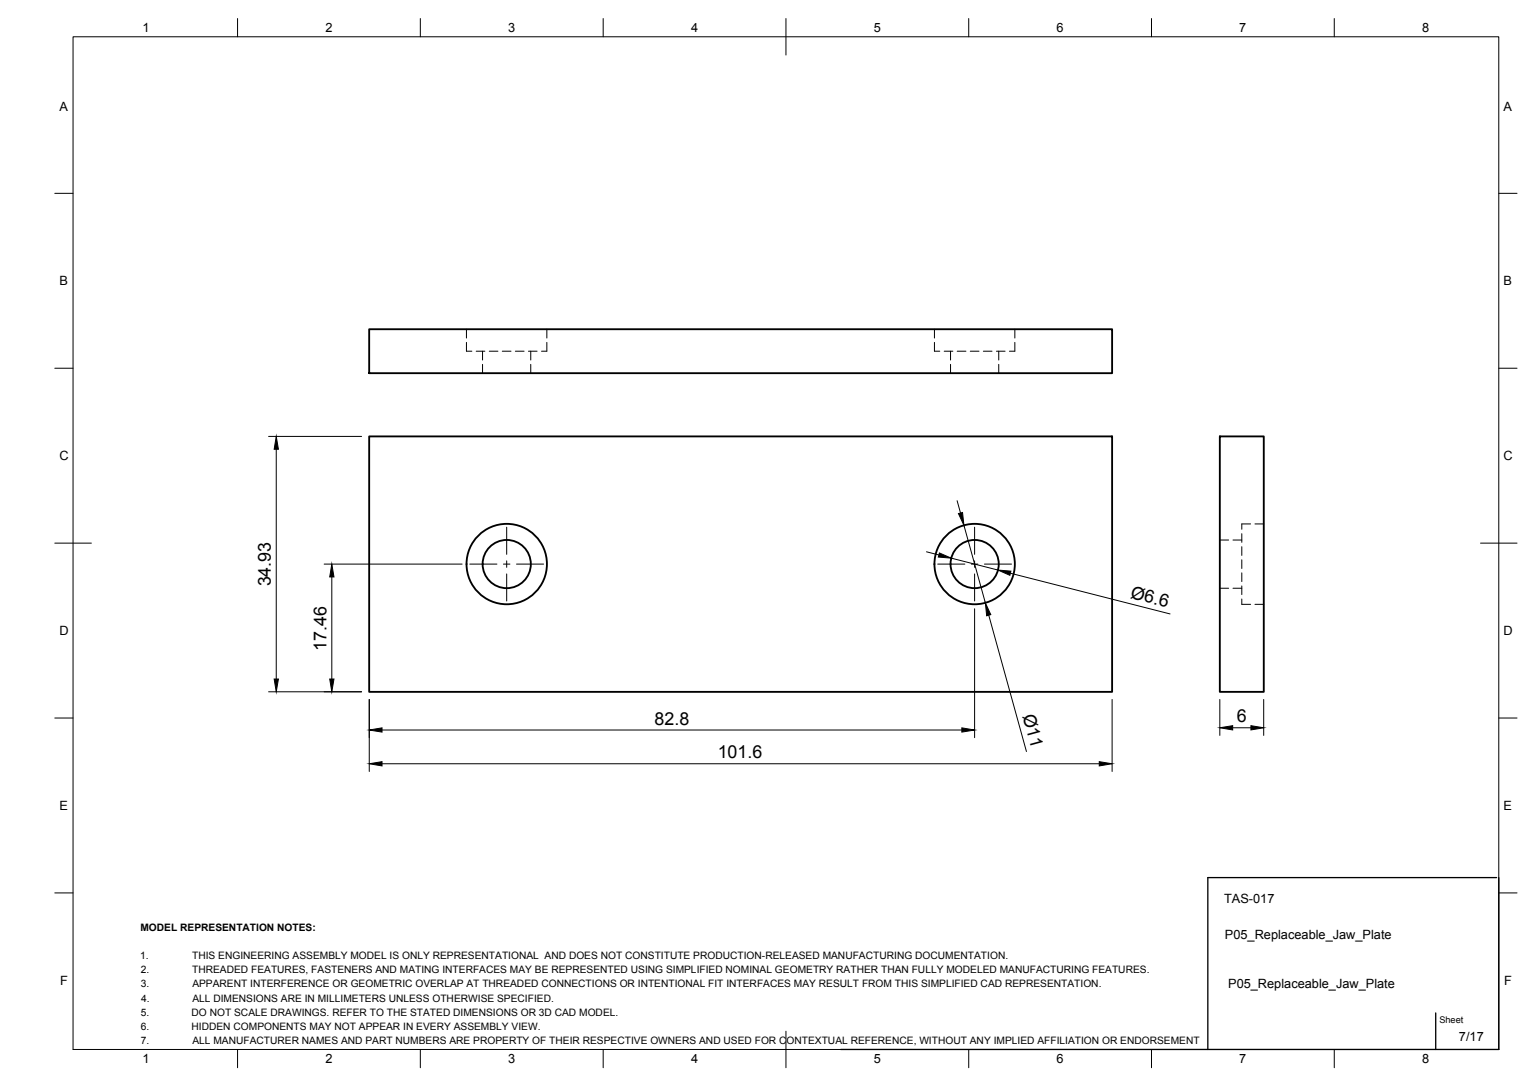
ISO-10303-21;
HEADER;
/* Generated by software containing ST-Developer
 * from STEP Tools, Inc. (www.steptools.com) 
 */

FILE_DESCRIPTION(
/* description */ ('STEP AP203'),
/* implementation_level */ '2;1');

FILE_NAME(
/* name */ 'P05_Replaceable_Jaw_Plate.step',
/* time_stamp */ '2026-11-15T15:04:01-08:00',
/* author */ (''),
/* organization */ (''),
/* preprocessor_version */ 'ST-DEVELOPER v20.2',
/* originating_system */ 'Autodesk Translation Framework v15.17.0.0',
/* authorisation */ '');

FILE_SCHEMA (('AUTOMOTIVE_DESIGN { 1 0 10303 214 3 1 1 }'));
ENDSEC;

DATA;
#10=MECHANICAL_DESIGN_GEOMETRIC_PRESENTATION_REPRESENTATION('',(#296),#16598);
#218=SHAPE_REPRESENTATION_RELATIONSHIP('SRR','None',#16712,#242);
#242=ADVANCED_BREP_SHAPE_REPRESENTATION('',(#266),#16588);
#266=MANIFOLD_SOLID_BREP('Body1',#9801);
#296=STYLED_ITEM('',(#16834),#266);
#362=FACE_BOUND('',#1777,.T.);
#363=FACE_BOUND('',#1778,.T.);
#364=FACE_BOUND('',#1780,.T.);
#365=FACE_BOUND('',#1781,.T.);
#366=FACE_BOUND('',#1783,.T.);
#367=FACE_BOUND('',#1785,.T.);
#633=PLANE('',#10459);
#634=PLANE('',#10460);
#635=PLANE('',#10461);
#636=PLANE('',#10462);
#637=PLANE('',#10463);
#638=PLANE('',#10464);
#639=PLANE('',#10465);
#640=PLANE('',#10466);
#1161=FACE_OUTER_BOUND('',#1768,.T.);
#1162=FACE_OUTER_BOUND('',#1769,.T.);
#1163=FACE_OUTER_BOUND('',#1770,.T.);
#1164=FACE_OUTER_BOUND('',#1771,.T.);
#1165=FACE_OUTER_BOUND('',#1772,.T.);
#1166=FACE_OUTER_BOUND('',#1773,.T.);
#1167=FACE_OUTER_BOUND('',#1774,.T.);
#1168=FACE_OUTER_BOUND('',#1775,.T.);
#1169=FACE_OUTER_BOUND('',#1776,.T.);
#1170=FACE_OUTER_BOUND('',#1779,.T.);
#1171=FACE_OUTER_BOUND('',#1782,.T.);
#1172=FACE_OUTER_BOUND('',#1784,.T.);
#1768=EDGE_LOOP('',(#7767,#7768,#7769,#7770));
#1769=EDGE_LOOP('',(#7771,#7772,#7773,#7774));
#1770=EDGE_LOOP('',(#7775,#7776,#7777,#7778));
#1771=EDGE_LOOP('',(#7779,#7780,#7781,#7782));
#1772=EDGE_LOOP('',(#7783,#7784,#7785,#7786));
#1773=EDGE_LOOP('',(#7787,#7788,#7789,#7790));
#1774=EDGE_LOOP('',(#7791,#7792,#7793,#7794));
#1775=EDGE_LOOP('',(#7795,#7796,#7797,#7798));
#1776=EDGE_LOOP('',(#7799,#7800,#7801,#7802));
#1777=EDGE_LOOP('',(#7803));
#1778=EDGE_LOOP('',(#7804));
#1779=EDGE_LOOP('',(#7805,#7806,#7807,#7808));
#1780=EDGE_LOOP('',(#7809));
#1781=EDGE_LOOP('',(#7810));
#1782=EDGE_LOOP('',(#7811));
#1783=EDGE_LOOP('',(#7812));
#1784=EDGE_LOOP('',(#7813));
#1785=EDGE_LOOP('',(#7814));
#2610=LINE('',#15029,#3658);
#2611=LINE('',#15035,#3659);
#2612=LINE('',#15041,#3660);
#2613=LINE('',#15047,#3661);
#2614=LINE('',#15052,#3662);
#2615=LINE('',#15054,#3663);
#2616=LINE('',#15056,#3664);
#2617=LINE('',#15057,#3665);
#2618=LINE('',#15060,#3666);
#2619=LINE('',#15062,#3667);
#2620=LINE('',#15063,#3668);
#2621=LINE('',#15066,#3669);
#2622=LINE('',#15068,#3670);
#2623=LINE('',#15069,#3671);
#2624=LINE('',#15071,#3672);
#2625=LINE('',#15072,#3673);
#3658=VECTOR('',#12148,5.50000000000001);
#3659=VECTOR('',#12155,5.50000000000001);
#3660=VECTOR('',#12162,3.3);
#3661=VECTOR('',#12169,3.3);
#3662=VECTOR('',#12174,1000.);
#3663=VECTOR('',#12175,1000.);
#3664=VECTOR('',#12176,1000.);
#3665=VECTOR('',#12177,1000.);
#3666=VECTOR('',#12180,1000.);
#3667=VECTOR('',#12181,1000.);
#3668=VECTOR('',#12182,1000.);
#3669=VECTOR('',#12185,1000.);
#3670=VECTOR('',#12186,1000.);
#3671=VECTOR('',#12187,1000.);
#3672=VECTOR('',#12190,1000.);
#3673=VECTOR('',#12191,1000.);
#4328=CIRCLE('',#10448,5.50000000000001);
#4329=CIRCLE('',#10449,5.50000000000001);
#4330=CIRCLE('',#10451,5.50000000000001);
#4331=CIRCLE('',#10452,5.50000000000001);
#4332=CIRCLE('',#10454,3.3);
#4333=CIRCLE('',#10455,3.3);
#4334=CIRCLE('',#10457,3.3);
#4335=CIRCLE('',#10458,3.3);
#4844=VERTEX_POINT('',#15026);
#4845=VERTEX_POINT('',#15028);
#4846=VERTEX_POINT('',#15032);
#4847=VERTEX_POINT('',#15034);
#4848=VERTEX_POINT('',#15038);
#4849=VERTEX_POINT('',#15040);
#4850=VERTEX_POINT('',#15044);
#4851=VERTEX_POINT('',#15046);
#4852=VERTEX_POINT('',#15050);
#4853=VERTEX_POINT('',#15051);
#4854=VERTEX_POINT('',#15053);
#4855=VERTEX_POINT('',#15055);
#4856=VERTEX_POINT('',#15059);
#4857=VERTEX_POINT('',#15061);
#4858=VERTEX_POINT('',#15065);
#4859=VERTEX_POINT('',#15067);
#5896=EDGE_CURVE('',#4844,#4844,#4328,.T.);
#5897=EDGE_CURVE('',#4844,#4845,#2610,.T.);
#5898=EDGE_CURVE('',#4845,#4845,#4329,.T.);
#5899=EDGE_CURVE('',#4846,#4846,#4330,.T.);
#5900=EDGE_CURVE('',#4846,#4847,#2611,.T.);
#5901=EDGE_CURVE('',#4847,#4847,#4331,.T.);
#5902=EDGE_CURVE('',#4848,#4848,#4332,.T.);
#5903=EDGE_CURVE('',#4848,#4849,#2612,.T.);
#5904=EDGE_CURVE('',#4849,#4849,#4333,.T.);
#5905=EDGE_CURVE('',#4850,#4850,#4334,.T.);
#5906=EDGE_CURVE('',#4850,#4851,#2613,.T.);
#5907=EDGE_CURVE('',#4851,#4851,#4335,.T.);
#5908=EDGE_CURVE('',#4852,#4853,#2614,.T.);
#5909=EDGE_CURVE('',#4854,#4853,#2615,.T.);
#5910=EDGE_CURVE('',#4855,#4854,#2616,.T.);
#5911=EDGE_CURVE('',#4855,#4852,#2617,.T.);
#5912=EDGE_CURVE('',#4853,#4856,#2618,.T.);
#5913=EDGE_CURVE('',#4857,#4856,#2619,.T.);
#5914=EDGE_CURVE('',#4854,#4857,#2620,.T.);
#5915=EDGE_CURVE('',#4856,#4858,#2621,.T.);
#5916=EDGE_CURVE('',#4859,#4858,#2622,.T.);
#5917=EDGE_CURVE('',#4857,#4859,#2623,.T.);
#5918=EDGE_CURVE('',#4858,#4852,#2624,.T.);
#5919=EDGE_CURVE('',#4859,#4855,#2625,.T.);
#7767=ORIENTED_EDGE('',*,*,#5896,.T.);
#7768=ORIENTED_EDGE('',*,*,#5897,.T.);
#7769=ORIENTED_EDGE('',*,*,#5898,.F.);
#7770=ORIENTED_EDGE('',*,*,#5897,.F.);
#7771=ORIENTED_EDGE('',*,*,#5899,.T.);
#7772=ORIENTED_EDGE('',*,*,#5900,.T.);
#7773=ORIENTED_EDGE('',*,*,#5901,.F.);
#7774=ORIENTED_EDGE('',*,*,#5900,.F.);
#7775=ORIENTED_EDGE('',*,*,#5902,.F.);
#7776=ORIENTED_EDGE('',*,*,#5903,.T.);
#7777=ORIENTED_EDGE('',*,*,#5904,.F.);
#7778=ORIENTED_EDGE('',*,*,#5903,.F.);
#7779=ORIENTED_EDGE('',*,*,#5905,.F.);
#7780=ORIENTED_EDGE('',*,*,#5906,.T.);
#7781=ORIENTED_EDGE('',*,*,#5907,.F.);
#7782=ORIENTED_EDGE('',*,*,#5906,.F.);
#7783=ORIENTED_EDGE('',*,*,#5908,.T.);
#7784=ORIENTED_EDGE('',*,*,#5909,.F.);
#7785=ORIENTED_EDGE('',*,*,#5910,.F.);
#7786=ORIENTED_EDGE('',*,*,#5911,.T.);
#7787=ORIENTED_EDGE('',*,*,#5912,.T.);
#7788=ORIENTED_EDGE('',*,*,#5913,.F.);
#7789=ORIENTED_EDGE('',*,*,#5914,.F.);
#7790=ORIENTED_EDGE('',*,*,#5909,.T.);
#7791=ORIENTED_EDGE('',*,*,#5915,.T.);
#7792=ORIENTED_EDGE('',*,*,#5916,.F.);
#7793=ORIENTED_EDGE('',*,*,#5917,.F.);
#7794=ORIENTED_EDGE('',*,*,#5913,.T.);
#7795=ORIENTED_EDGE('',*,*,#5918,.T.);
#7796=ORIENTED_EDGE('',*,*,#5911,.F.);
#7797=ORIENTED_EDGE('',*,*,#5919,.F.);
#7798=ORIENTED_EDGE('',*,*,#5916,.T.);
#7799=ORIENTED_EDGE('',*,*,#5910,.T.);
#7800=ORIENTED_EDGE('',*,*,#5914,.T.);
#7801=ORIENTED_EDGE('',*,*,#5917,.T.);
#7802=ORIENTED_EDGE('',*,*,#5919,.T.);
#7803=ORIENTED_EDGE('',*,*,#5902,.T.);
#7804=ORIENTED_EDGE('',*,*,#5905,.T.);
#7805=ORIENTED_EDGE('',*,*,#5908,.F.);
#7806=ORIENTED_EDGE('',*,*,#5918,.F.);
#7807=ORIENTED_EDGE('',*,*,#5915,.F.);
#7808=ORIENTED_EDGE('',*,*,#5912,.F.);
#7809=ORIENTED_EDGE('',*,*,#5901,.T.);
#7810=ORIENTED_EDGE('',*,*,#5898,.T.);
#7811=ORIENTED_EDGE('',*,*,#5899,.F.);
#7812=ORIENTED_EDGE('',*,*,#5904,.T.);
#7813=ORIENTED_EDGE('',*,*,#5896,.F.);
#7814=ORIENTED_EDGE('',*,*,#5907,.T.);
#9215=CYLINDRICAL_SURFACE('',#10447,5.50000000000001);
#9216=CYLINDRICAL_SURFACE('',#10450,5.50000000000001);
#9217=CYLINDRICAL_SURFACE('',#10453,3.3);
#9218=CYLINDRICAL_SURFACE('',#10456,3.3);
#9486=ADVANCED_FACE('',(#1161),#9215,.F.);
#9487=ADVANCED_FACE('',(#1162),#9216,.F.);
#9488=ADVANCED_FACE('',(#1163),#9217,.F.);
#9489=ADVANCED_FACE('',(#1164),#9218,.F.);
#9490=ADVANCED_FACE('',(#1165),#633,.F.);
#9491=ADVANCED_FACE('',(#1166),#634,.F.);
#9492=ADVANCED_FACE('',(#1167),#635,.F.);
#9493=ADVANCED_FACE('',(#1168),#636,.F.);
#9494=ADVANCED_FACE('',(#1169,#362,#363),#637,.T.);
#9495=ADVANCED_FACE('',(#1170,#364,#365),#638,.F.);
#9496=ADVANCED_FACE('',(#1171,#366),#639,.F.);
#9497=ADVANCED_FACE('',(#1172,#367),#640,.F.);
#9801=CLOSED_SHELL('',(#9486,#9487,#9488,#9489,#9490,#9491,#9492,#9493,
#9494,#9495,#9496,#9497));
#10446=AXIS2_PLACEMENT_3D('',#15024,#12142,#12143);
#10447=AXIS2_PLACEMENT_3D('',#15025,#12144,#12145);
#10448=AXIS2_PLACEMENT_3D('',#15027,#12146,#12147);
#10449=AXIS2_PLACEMENT_3D('',#15030,#12149,#12150);
#10450=AXIS2_PLACEMENT_3D('',#15031,#12151,#12152);
#10451=AXIS2_PLACEMENT_3D('',#15033,#12153,#12154);
#10452=AXIS2_PLACEMENT_3D('',#15036,#12156,#12157);
#10453=AXIS2_PLACEMENT_3D('',#15037,#12158,#12159);
#10454=AXIS2_PLACEMENT_3D('',#15039,#12160,#12161);
#10455=AXIS2_PLACEMENT_3D('',#15042,#12163,#12164);
#10456=AXIS2_PLACEMENT_3D('',#15043,#12165,#12166);
#10457=AXIS2_PLACEMENT_3D('',#15045,#12167,#12168);
#10458=AXIS2_PLACEMENT_3D('',#15048,#12170,#12171);
#10459=AXIS2_PLACEMENT_3D('',#15049,#12172,#12173);
#10460=AXIS2_PLACEMENT_3D('',#15058,#12178,#12179);
#10461=AXIS2_PLACEMENT_3D('',#15064,#12183,#12184);
#10462=AXIS2_PLACEMENT_3D('',#15070,#12188,#12189);
#10463=AXIS2_PLACEMENT_3D('',#15073,#12192,#12193);
#10464=AXIS2_PLACEMENT_3D('',#15074,#12194,#12195);
#10465=AXIS2_PLACEMENT_3D('',#15075,#12196,#12197);
#10466=AXIS2_PLACEMENT_3D('',#15076,#12198,#12199);
#12142=DIRECTION('axis',(0.,0.,1.));
#12143=DIRECTION('refdir',(1.,0.,0.));
#12144=DIRECTION('center_axis',(0.,-1.,0.));
#12145=DIRECTION('ref_axis',(0.,0.,-1.));
#12146=DIRECTION('center_axis',(0.,1.,0.));
#12147=DIRECTION('ref_axis',(0.,0.,1.));
#12148=DIRECTION('',(0.,-1.,0.));
#12149=DIRECTION('center_axis',(0.,1.,0.));
#12150=DIRECTION('ref_axis',(0.,0.,1.));
#12151=DIRECTION('center_axis',(0.,-1.,0.));
#12152=DIRECTION('ref_axis',(0.,0.,-1.));
#12153=DIRECTION('center_axis',(0.,1.,0.));
#12154=DIRECTION('ref_axis',(0.,0.,1.));
#12155=DIRECTION('',(0.,-1.,0.));
#12156=DIRECTION('center_axis',(0.,1.,0.));
#12157=DIRECTION('ref_axis',(0.,0.,1.));
#12158=DIRECTION('center_axis',(0.,-1.,0.));
#12159=DIRECTION('ref_axis',(0.,0.,-1.));
#12160=DIRECTION('center_axis',(0.,-1.,0.));
#12161=DIRECTION('ref_axis',(0.,0.,1.));
#12162=DIRECTION('',(0.,-1.,0.));
#12163=DIRECTION('center_axis',(0.,1.,0.));
#12164=DIRECTION('ref_axis',(0.,0.,1.));
#12165=DIRECTION('center_axis',(0.,-1.,0.));
#12166=DIRECTION('ref_axis',(0.,0.,-1.));
#12167=DIRECTION('center_axis',(0.,-1.,0.));
#12168=DIRECTION('ref_axis',(0.,0.,1.));
#12169=DIRECTION('',(0.,-1.,0.));
#12170=DIRECTION('center_axis',(0.,1.,0.));
#12171=DIRECTION('ref_axis',(0.,0.,1.));
#12172=DIRECTION('center_axis',(-1.,0.,0.));
#12173=DIRECTION('ref_axis',(0.,0.,1.));
#12174=DIRECTION('',(0.,0.,-1.));
#12175=DIRECTION('',(0.,-1.,0.));
#12176=DIRECTION('',(0.,0.,-1.));
#12177=DIRECTION('',(0.,-1.,0.));
#12178=DIRECTION('center_axis',(0.,0.,1.));
#12179=DIRECTION('ref_axis',(1.,0.,0.));
#12180=DIRECTION('',(-1.,0.,0.));
#12181=DIRECTION('',(0.,-1.,0.));
#12182=DIRECTION('',(-1.,0.,0.));
#12183=DIRECTION('center_axis',(1.,0.,0.));
#12184=DIRECTION('ref_axis',(0.,0.,-1.));
#12185=DIRECTION('',(0.,0.,1.));
#12186=DIRECTION('',(0.,-1.,0.));
#12187=DIRECTION('',(0.,0.,1.));
#12188=DIRECTION('center_axis',(0.,0.,-1.));
#12189=DIRECTION('ref_axis',(-1.,0.,0.));
#12190=DIRECTION('',(1.,0.,0.));
#12191=DIRECTION('',(1.,0.,0.));
#12192=DIRECTION('center_axis',(0.,1.,0.));
#12193=DIRECTION('ref_axis',(0.,0.,1.));
#12194=DIRECTION('center_axis',(0.,1.,0.));
#12195=DIRECTION('ref_axis',(0.,0.,1.));
#12196=DIRECTION('center_axis',(0.,1.,0.));
#12197=DIRECTION('ref_axis',(0.,0.,1.));
#12198=DIRECTION('center_axis',(0.,1.,0.));
#12199=DIRECTION('ref_axis',(0.,0.,1.));
#15024=CARTESIAN_POINT('',(0.,0.,0.));
#15025=CARTESIAN_POINT('Origin',(32.,3.,115.8875));
#15026=CARTESIAN_POINT('',(32.,3.,121.3875));
#15027=CARTESIAN_POINT('Origin',(32.,3.,115.8875));
#15028=CARTESIAN_POINT('',(32.,0.,121.3875));
#15029=CARTESIAN_POINT('',(32.,3.,121.3875));
#15030=CARTESIAN_POINT('Origin',(32.,0.,115.8875));
#15031=CARTESIAN_POINT('Origin',(-32.,3.,115.8875));
#15032=CARTESIAN_POINT('',(-32.,3.,121.3875));
#15033=CARTESIAN_POINT('Origin',(-32.,3.,115.8875));
#15034=CARTESIAN_POINT('',(-32.,0.,121.3875));
#15035=CARTESIAN_POINT('',(-32.,3.,121.3875));
#15036=CARTESIAN_POINT('Origin',(-32.,0.,115.8875));
#15037=CARTESIAN_POINT('Origin',(-32.,7.,115.8875));
#15038=CARTESIAN_POINT('',(-32.,6.,119.1875));
#15039=CARTESIAN_POINT('Origin',(-32.,6.,115.8875));
#15040=CARTESIAN_POINT('',(-32.,3.,119.1875));
#15041=CARTESIAN_POINT('',(-32.,7.,119.1875));
#15042=CARTESIAN_POINT('Origin',(-32.,3.,115.8875));
#15043=CARTESIAN_POINT('Origin',(32.,7.,115.8875));
#15044=CARTESIAN_POINT('',(32.,6.,119.1875));
#15045=CARTESIAN_POINT('Origin',(32.,6.,115.8875));
#15046=CARTESIAN_POINT('',(32.,3.,119.1875));
#15047=CARTESIAN_POINT('',(32.,7.,119.1875));
#15048=CARTESIAN_POINT('Origin',(32.,3.,115.8875));
#15049=CARTESIAN_POINT('Origin',(50.8,6.,98.425));
#15050=CARTESIAN_POINT('',(50.8,0.,133.35));
#15051=CARTESIAN_POINT('',(50.8,0.,98.425));
#15052=CARTESIAN_POINT('',(50.8,0.,98.425));
#15053=CARTESIAN_POINT('',(50.8,6.,98.425));
#15054=CARTESIAN_POINT('',(50.8,6.,98.425));
#15055=CARTESIAN_POINT('',(50.8,6.,133.35));
#15056=CARTESIAN_POINT('',(50.8,6.,98.425));
#15057=CARTESIAN_POINT('',(50.8,6.,133.35));
#15058=CARTESIAN_POINT('Origin',(-50.8,6.,98.425));
#15059=CARTESIAN_POINT('',(-50.8,0.,98.425));
#15060=CARTESIAN_POINT('',(-50.8,0.,98.425));
#15061=CARTESIAN_POINT('',(-50.8,6.,98.425));
#15062=CARTESIAN_POINT('',(-50.8,6.,98.425));
#15063=CARTESIAN_POINT('',(-50.8,6.,98.425));
#15064=CARTESIAN_POINT('Origin',(-50.8,6.,98.425));
#15065=CARTESIAN_POINT('',(-50.8,0.,133.35));
#15066=CARTESIAN_POINT('',(-50.8,0.,98.425));
#15067=CARTESIAN_POINT('',(-50.8,6.,133.35));
#15068=CARTESIAN_POINT('',(-50.8,6.,133.35));
#15069=CARTESIAN_POINT('',(-50.8,6.,98.425));
#15070=CARTESIAN_POINT('Origin',(-50.8,6.,133.35));
#15071=CARTESIAN_POINT('',(-50.8,0.,133.35));
#15072=CARTESIAN_POINT('',(-50.8,6.,133.35));
#15073=CARTESIAN_POINT('Origin',(0.,6.,0.));
#15074=CARTESIAN_POINT('Origin',(0.,0.,0.));
#15075=CARTESIAN_POINT('Origin',(-32.,3.,115.8875));
#15076=CARTESIAN_POINT('Origin',(32.,3.,115.8875));
#16562=UNCERTAINTY_MEASURE_WITH_UNIT(LENGTH_MEASURE(0.01),#16599,
'DISTANCE_ACCURACY_VALUE',
'Maximum model space distance between geometric entities at asserted c
onnectivities');
#16572=UNCERTAINTY_MEASURE_WITH_UNIT(LENGTH_MEASURE(0.01),#16599,
'DISTANCE_ACCURACY_VALUE',
'Maximum model space distance between geometric entities at asserted c
onnectivities');
#16588=(
GEOMETRIC_REPRESENTATION_CONTEXT(3)
GLOBAL_UNCERTAINTY_ASSIGNED_CONTEXT((#16562))
GLOBAL_UNIT_ASSIGNED_CONTEXT((#16599,#16601,#16602))
REPRESENTATION_CONTEXT('','3D')
);
#16598=(
GEOMETRIC_REPRESENTATION_CONTEXT(3)
GLOBAL_UNCERTAINTY_ASSIGNED_CONTEXT((#16572))
GLOBAL_UNIT_ASSIGNED_CONTEXT((#16599,#16601,#16602))
REPRESENTATION_CONTEXT('','3D')
);
#16599=(
LENGTH_UNIT()
NAMED_UNIT(*)
SI_UNIT(.MILLI.,.METRE.)
);
#16601=(
NAMED_UNIT(*)
PLANE_ANGLE_UNIT()
SI_UNIT($,.RADIAN.)
);
#16602=(
NAMED_UNIT(*)
SI_UNIT($,.STERADIAN.)
SOLID_ANGLE_UNIT()
);
#16618=SHAPE_DEFINITION_REPRESENTATION(#16643,#16712);
#16643=PRODUCT_DEFINITION_SHAPE('',$,#16738);
#16712=SHAPE_REPRESENTATION('',(#10446),#16588);
#16722=PRODUCT_DEFINITION_CONTEXT('part definition',#16799,'design');
#16738=PRODUCT_DEFINITION('P05_Replaceable_Jaw_Plate',
'P05_Replaceable_Jaw_Plate',#16763,#16722);
#16763=PRODUCT_DEFINITION_FORMATION('',$,#16816);
#16799=APPLICATION_CONTEXT(
'Core Data for Automotive Mechanical Design Process');
#16800=PRODUCT_CONTEXT('part definition',#16799,'mechanical');
#16816=PRODUCT('P05_Replaceable_Jaw_Plate','P05_Replaceable_Jaw_Plate',
$,(#16800));
#16834=PRESENTATION_STYLE_ASSIGNMENT((#16843));
#16843=SURFACE_STYLE_USAGE(.BOTH.,#16852);
#16852=SURFACE_SIDE_STYLE('',(#16861));
#16861=SURFACE_STYLE_FILL_AREA(#16870);
#16870=FILL_AREA_STYLE('Light Blue',(#16879));
#16879=FILL_AREA_STYLE_COLOUR('Light Blue',#16888);
#16888=COLOUR_RGB('Light Blue',0.67843137254902,0.847058823529412,0.901960784313726);
ENDSEC;
END-ISO-10303-21;
